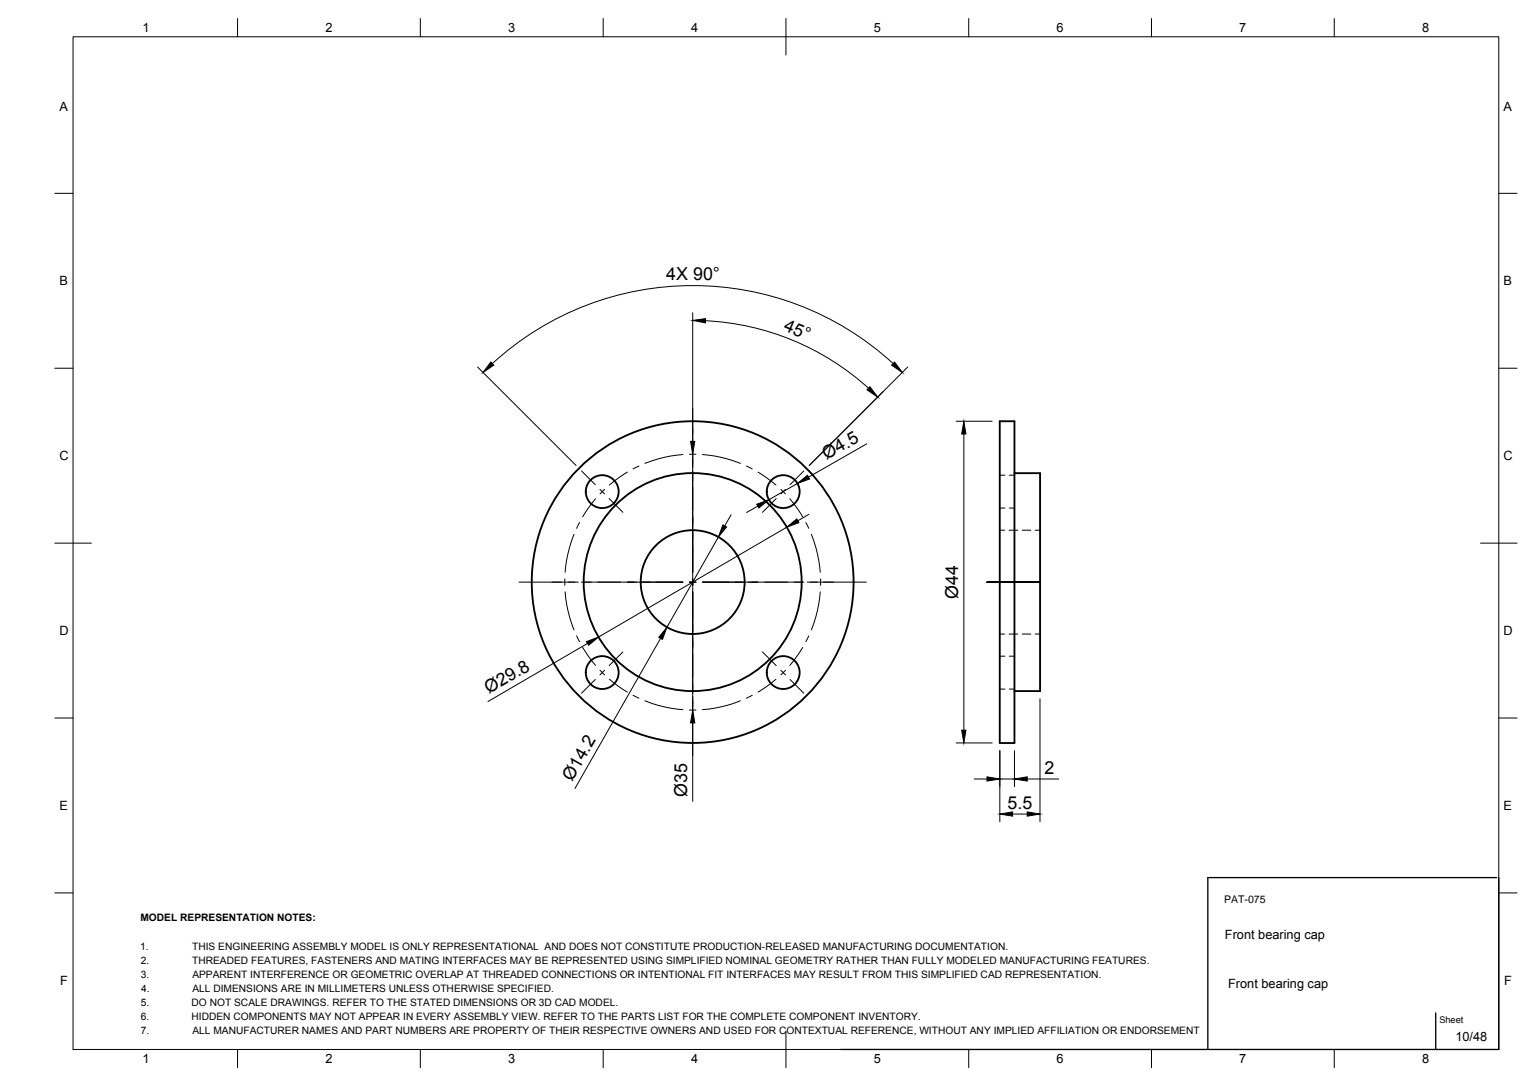
ISO-10303-21;
HEADER;
/* Generated by software containing ST-Developer
 * from STEP Tools, Inc. (www.steptools.com) 
 */

FILE_DESCRIPTION(
/* description */ ('Over-Centre Plunger Toggle Clamp on Slotted Fixture Frame'),
/* implementation_level */ '2;1');

FILE_NAME(
/* name */ 
'Front bearing cap.step',
/* time_stamp */ '2026-10-28T03:23:24-07:00',
/* author */ (''),
/* organization */ (''),
/* preprocessor_version */ 'ST-DEVELOPER v20.2',
/* originating_system */ 'Autodesk Translation Framework v15.17.0.0',
/* authorisation */ '');

FILE_SCHEMA (('AUTOMOTIVE_DESIGN { 1 0 10303 214 3 1 1 }'));
ENDSEC;

DATA;
#10=MECHANICAL_DESIGN_GEOMETRIC_PRESENTATION_REPRESENTATION('',(#518),#15212);
#434=SHAPE_REPRESENTATION_RELATIONSHIP('SRR','None',#15408,#476);
#476=ADVANCED_BREP_SHAPE_REPRESENTATION('',(#569),#15170);
#518=STYLED_ITEM('',(#15719),#569);
#569=MANIFOLD_SOLID_BREP('Body1',#8250);
#671=FACE_BOUND('',#1717,.T.);
#672=FACE_BOUND('',#1721,.T.);
#673=FACE_BOUND('',#1722,.T.);
#674=FACE_BOUND('',#1723,.T.);
#675=FACE_BOUND('',#1724,.T.);
#676=FACE_BOUND('',#1725,.T.);
#677=FACE_BOUND('',#1727,.T.);
#678=FACE_BOUND('',#1728,.T.);
#679=FACE_BOUND('',#1729,.T.);
#680=FACE_BOUND('',#1730,.T.);
#681=FACE_BOUND('',#1731,.T.);
#827=PLANE('',#8932);
#828=PLANE('',#8939);
#829=PLANE('',#8940);
#1165=FACE_OUTER_BOUND('',#1711,.T.);
#1166=FACE_OUTER_BOUND('',#1712,.T.);
#1167=FACE_OUTER_BOUND('',#1713,.T.);
#1168=FACE_OUTER_BOUND('',#1714,.T.);
#1169=FACE_OUTER_BOUND('',#1715,.T.);
#1170=FACE_OUTER_BOUND('',#1716,.T.);
#1171=FACE_OUTER_BOUND('',#1718,.T.);
#1172=FACE_OUTER_BOUND('',#1719,.T.);
#1173=FACE_OUTER_BOUND('',#1720,.T.);
#1174=FACE_OUTER_BOUND('',#1726,.T.);
#1711=EDGE_LOOP('',(#5941,#5942,#5943,#5944));
#1712=EDGE_LOOP('',(#5945,#5946,#5947,#5948));
#1713=EDGE_LOOP('',(#5949,#5950,#5951,#5952));
#1714=EDGE_LOOP('',(#5953,#5954,#5955,#5956));
#1715=EDGE_LOOP('',(#5957,#5958,#5959,#5960));
#1716=EDGE_LOOP('',(#5961));
#1717=EDGE_LOOP('',(#5962));
#1718=EDGE_LOOP('',(#5963,#5964,#5965,#5966));
#1719=EDGE_LOOP('',(#5967,#5968,#5969,#5970));
#1720=EDGE_LOOP('',(#5971));
#1721=EDGE_LOOP('',(#5972));
#1722=EDGE_LOOP('',(#5973));
#1723=EDGE_LOOP('',(#5974));
#1724=EDGE_LOOP('',(#5975));
#1725=EDGE_LOOP('',(#5976));
#1726=EDGE_LOOP('',(#5977));
#1727=EDGE_LOOP('',(#5978));
#1728=EDGE_LOOP('',(#5979));
#1729=EDGE_LOOP('',(#5980));
#1730=EDGE_LOOP('',(#5981));
#1731=EDGE_LOOP('',(#5982));
#2349=LINE('',#12766,#2979);
#2350=LINE('',#12772,#2980);
#2351=LINE('',#12778,#2981);
#2352=LINE('',#12784,#2982);
#2353=LINE('',#12790,#2983);
#2354=LINE('',#12797,#2984);
#2355=LINE('',#12803,#2985);
#2979=VECTOR('',#10184,0.225);
#2980=VECTOR('',#10191,0.225);
#2981=VECTOR('',#10198,0.225);
#2982=VECTOR('',#10205,0.225);
#2983=VECTOR('',#10212,1.49);
#2984=VECTOR('',#10221,0.71);
#2985=VECTOR('',#10228,2.2);
#3559=CIRCLE('',#8918,0.225);
#3560=CIRCLE('',#8919,0.225);
#3561=CIRCLE('',#8921,0.225);
#3562=CIRCLE('',#8922,0.225);
#3563=CIRCLE('',#8924,0.225);
#3564=CIRCLE('',#8925,0.225);
#3565=CIRCLE('',#8927,0.225);
#3566=CIRCLE('',#8928,0.225);
#3567=CIRCLE('',#8930,1.49);
#3568=CIRCLE('',#8931,1.49);
#3569=CIRCLE('',#8933,0.71);
#3570=CIRCLE('',#8935,0.71);
#3571=CIRCLE('',#8937,2.2);
#3572=CIRCLE('',#8938,2.2);
#3983=VERTEX_POINT('',#12763);
#3984=VERTEX_POINT('',#12765);
#3985=VERTEX_POINT('',#12769);
#3986=VERTEX_POINT('',#12771);
#3987=VERTEX_POINT('',#12775);
#3988=VERTEX_POINT('',#12777);
#3989=VERTEX_POINT('',#12781);
#3990=VERTEX_POINT('',#12783);
#3991=VERTEX_POINT('',#12787);
#3992=VERTEX_POINT('',#12789);
#3993=VERTEX_POINT('',#12793);
#3994=VERTEX_POINT('',#12796);
#3995=VERTEX_POINT('',#12800);
#3996=VERTEX_POINT('',#12802);
#4731=EDGE_CURVE('',#3983,#3983,#3559,.T.);
#4732=EDGE_CURVE('',#3983,#3984,#2349,.T.);
#4733=EDGE_CURVE('',#3984,#3984,#3560,.T.);
#4734=EDGE_CURVE('',#3985,#3985,#3561,.T.);
#4735=EDGE_CURVE('',#3985,#3986,#2350,.T.);
#4736=EDGE_CURVE('',#3986,#3986,#3562,.T.);
#4737=EDGE_CURVE('',#3987,#3987,#3563,.T.);
#4738=EDGE_CURVE('',#3987,#3988,#2351,.T.);
#4739=EDGE_CURVE('',#3988,#3988,#3564,.T.);
#4740=EDGE_CURVE('',#3989,#3989,#3565,.T.);
#4741=EDGE_CURVE('',#3989,#3990,#2352,.T.);
#4742=EDGE_CURVE('',#3990,#3990,#3566,.T.);
#4743=EDGE_CURVE('',#3991,#3991,#3567,.T.);
#4744=EDGE_CURVE('',#3991,#3992,#2353,.T.);
#4745=EDGE_CURVE('',#3992,#3992,#3568,.T.);
#4746=EDGE_CURVE('',#3993,#3993,#3569,.T.);
#4747=EDGE_CURVE('',#3993,#3994,#2354,.T.);
#4748=EDGE_CURVE('',#3994,#3994,#3570,.T.);
#4749=EDGE_CURVE('',#3995,#3995,#3571,.T.);
#4750=EDGE_CURVE('',#3995,#3996,#2355,.T.);
#4751=EDGE_CURVE('',#3996,#3996,#3572,.T.);
#5941=ORIENTED_EDGE('',*,*,#4731,.F.);
#5942=ORIENTED_EDGE('',*,*,#4732,.T.);
#5943=ORIENTED_EDGE('',*,*,#4733,.F.);
#5944=ORIENTED_EDGE('',*,*,#4732,.F.);
#5945=ORIENTED_EDGE('',*,*,#4734,.F.);
#5946=ORIENTED_EDGE('',*,*,#4735,.T.);
#5947=ORIENTED_EDGE('',*,*,#4736,.F.);
#5948=ORIENTED_EDGE('',*,*,#4735,.F.);
#5949=ORIENTED_EDGE('',*,*,#4737,.F.);
#5950=ORIENTED_EDGE('',*,*,#4738,.T.);
#5951=ORIENTED_EDGE('',*,*,#4739,.F.);
#5952=ORIENTED_EDGE('',*,*,#4738,.F.);
#5953=ORIENTED_EDGE('',*,*,#4740,.F.);
#5954=ORIENTED_EDGE('',*,*,#4741,.T.);
#5955=ORIENTED_EDGE('',*,*,#4742,.F.);
#5956=ORIENTED_EDGE('',*,*,#4741,.F.);
#5957=ORIENTED_EDGE('',*,*,#4743,.F.);
#5958=ORIENTED_EDGE('',*,*,#4744,.T.);
#5959=ORIENTED_EDGE('',*,*,#4745,.F.);
#5960=ORIENTED_EDGE('',*,*,#4744,.F.);
#5961=ORIENTED_EDGE('',*,*,#4743,.T.);
#5962=ORIENTED_EDGE('',*,*,#4746,.T.);
#5963=ORIENTED_EDGE('',*,*,#4746,.F.);
#5964=ORIENTED_EDGE('',*,*,#4747,.T.);
#5965=ORIENTED_EDGE('',*,*,#4748,.T.);
#5966=ORIENTED_EDGE('',*,*,#4747,.F.);
#5967=ORIENTED_EDGE('',*,*,#4749,.F.);
#5968=ORIENTED_EDGE('',*,*,#4750,.T.);
#5969=ORIENTED_EDGE('',*,*,#4751,.T.);
#5970=ORIENTED_EDGE('',*,*,#4750,.F.);
#5971=ORIENTED_EDGE('',*,*,#4749,.T.);
#5972=ORIENTED_EDGE('',*,*,#4745,.T.);
#5973=ORIENTED_EDGE('',*,*,#4742,.T.);
#5974=ORIENTED_EDGE('',*,*,#4739,.T.);
#5975=ORIENTED_EDGE('',*,*,#4736,.T.);
#5976=ORIENTED_EDGE('',*,*,#4733,.T.);
#5977=ORIENTED_EDGE('',*,*,#4751,.F.);
#5978=ORIENTED_EDGE('',*,*,#4748,.F.);
#5979=ORIENTED_EDGE('',*,*,#4740,.T.);
#5980=ORIENTED_EDGE('',*,*,#4737,.T.);
#5981=ORIENTED_EDGE('',*,*,#4734,.T.);
#5982=ORIENTED_EDGE('',*,*,#4731,.T.);
#7651=CYLINDRICAL_SURFACE('',#8917,0.225);
#7652=CYLINDRICAL_SURFACE('',#8920,0.225);
#7653=CYLINDRICAL_SURFACE('',#8923,0.225);
#7654=CYLINDRICAL_SURFACE('',#8926,0.225);
#7655=CYLINDRICAL_SURFACE('',#8929,1.49);
#7656=CYLINDRICAL_SURFACE('',#8934,0.71);
#7657=CYLINDRICAL_SURFACE('',#8936,2.2);
#7837=ADVANCED_FACE('',(#1165),#7651,.F.);
#7838=ADVANCED_FACE('',(#1166),#7652,.F.);
#7839=ADVANCED_FACE('',(#1167),#7653,.F.);
#7840=ADVANCED_FACE('',(#1168),#7654,.F.);
#7841=ADVANCED_FACE('',(#1169),#7655,.T.);
#7842=ADVANCED_FACE('',(#1170,#671),#827,.T.);
#7843=ADVANCED_FACE('',(#1171),#7656,.F.);
#7844=ADVANCED_FACE('',(#1172),#7657,.T.);
#7845=ADVANCED_FACE('',(#1173,#672,#673,#674,#675,#676),#828,.T.);
#7846=ADVANCED_FACE('',(#1174,#677,#678,#679,#680,#681),#829,.F.);
#8250=CLOSED_SHELL('',(#7837,#7838,#7839,#7840,#7841,#7842,#7843,#7844,
#7845,#7846));
#8916=AXIS2_PLACEMENT_3D('',#12761,#10178,#10179);
#8917=AXIS2_PLACEMENT_3D('',#12762,#10180,#10181);
#8918=AXIS2_PLACEMENT_3D('',#12764,#10182,#10183);
#8919=AXIS2_PLACEMENT_3D('',#12767,#10185,#10186);
#8920=AXIS2_PLACEMENT_3D('',#12768,#10187,#10188);
#8921=AXIS2_PLACEMENT_3D('',#12770,#10189,#10190);
#8922=AXIS2_PLACEMENT_3D('',#12773,#10192,#10193);
#8923=AXIS2_PLACEMENT_3D('',#12774,#10194,#10195);
#8924=AXIS2_PLACEMENT_3D('',#12776,#10196,#10197);
#8925=AXIS2_PLACEMENT_3D('',#12779,#10199,#10200);
#8926=AXIS2_PLACEMENT_3D('',#12780,#10201,#10202);
#8927=AXIS2_PLACEMENT_3D('',#12782,#10203,#10204);
#8928=AXIS2_PLACEMENT_3D('',#12785,#10206,#10207);
#8929=AXIS2_PLACEMENT_3D('',#12786,#10208,#10209);
#8930=AXIS2_PLACEMENT_3D('',#12788,#10210,#10211);
#8931=AXIS2_PLACEMENT_3D('',#12791,#10213,#10214);
#8932=AXIS2_PLACEMENT_3D('',#12792,#10215,#10216);
#8933=AXIS2_PLACEMENT_3D('',#12794,#10217,#10218);
#8934=AXIS2_PLACEMENT_3D('',#12795,#10219,#10220);
#8935=AXIS2_PLACEMENT_3D('',#12798,#10222,#10223);
#8936=AXIS2_PLACEMENT_3D('',#12799,#10224,#10225);
#8937=AXIS2_PLACEMENT_3D('',#12801,#10226,#10227);
#8938=AXIS2_PLACEMENT_3D('',#12804,#10229,#10230);
#8939=AXIS2_PLACEMENT_3D('',#12805,#10231,#10232);
#8940=AXIS2_PLACEMENT_3D('',#12806,#10233,#10234);
#10178=DIRECTION('axis',(0.,0.,1.));
#10179=DIRECTION('refdir',(1.,0.,0.));
#10180=DIRECTION('center_axis',(0.,1.,0.));
#10181=DIRECTION('ref_axis',(1.,0.,0.));
#10182=DIRECTION('center_axis',(0.,1.,0.));
#10183=DIRECTION('ref_axis',(1.,0.,0.));
#10184=DIRECTION('',(0.,1.,0.));
#10185=DIRECTION('center_axis',(0.,-1.,0.));
#10186=DIRECTION('ref_axis',(1.,0.,0.));
#10187=DIRECTION('center_axis',(0.,1.,0.));
#10188=DIRECTION('ref_axis',(1.,0.,0.));
#10189=DIRECTION('center_axis',(0.,1.,0.));
#10190=DIRECTION('ref_axis',(1.,0.,0.));
#10191=DIRECTION('',(0.,1.,0.));
#10192=DIRECTION('center_axis',(0.,-1.,0.));
#10193=DIRECTION('ref_axis',(1.,0.,0.));
#10194=DIRECTION('center_axis',(0.,1.,0.));
#10195=DIRECTION('ref_axis',(1.,0.,0.));
#10196=DIRECTION('center_axis',(0.,1.,0.));
#10197=DIRECTION('ref_axis',(1.,0.,0.));
#10198=DIRECTION('',(0.,1.,0.));
#10199=DIRECTION('center_axis',(0.,-1.,0.));
#10200=DIRECTION('ref_axis',(1.,0.,0.));
#10201=DIRECTION('center_axis',(0.,1.,0.));
#10202=DIRECTION('ref_axis',(1.,0.,0.));
#10203=DIRECTION('center_axis',(0.,1.,0.));
#10204=DIRECTION('ref_axis',(1.,0.,0.));
#10205=DIRECTION('',(0.,1.,0.));
#10206=DIRECTION('center_axis',(0.,-1.,0.));
#10207=DIRECTION('ref_axis',(1.,0.,0.));
#10208=DIRECTION('center_axis',(0.,1.,0.));
#10209=DIRECTION('ref_axis',(1.,0.,0.));
#10210=DIRECTION('center_axis',(0.,1.,0.));
#10211=DIRECTION('ref_axis',(1.,0.,0.));
#10212=DIRECTION('',(0.,-1.,0.));
#10213=DIRECTION('center_axis',(0.,-1.,0.));
#10214=DIRECTION('ref_axis',(1.,0.,0.));
#10215=DIRECTION('center_axis',(0.,1.,0.));
#10216=DIRECTION('ref_axis',(1.,0.,0.));
#10217=DIRECTION('center_axis',(0.,-1.,0.));
#10218=DIRECTION('ref_axis',(1.,0.,0.));
#10219=DIRECTION('center_axis',(0.,1.,0.));
#10220=DIRECTION('ref_axis',(1.,0.,0.));
#10221=DIRECTION('',(0.,-1.,0.));
#10222=DIRECTION('center_axis',(0.,-1.,0.));
#10223=DIRECTION('ref_axis',(1.,0.,0.));
#10224=DIRECTION('center_axis',(0.,1.,0.));
#10225=DIRECTION('ref_axis',(1.,0.,0.));
#10226=DIRECTION('center_axis',(0.,1.,0.));
#10227=DIRECTION('ref_axis',(1.,0.,0.));
#10228=DIRECTION('',(0.,-1.,0.));
#10229=DIRECTION('center_axis',(0.,1.,0.));
#10230=DIRECTION('ref_axis',(1.,0.,0.));
#10231=DIRECTION('center_axis',(0.,1.,0.));
#10232=DIRECTION('ref_axis',(1.,0.,0.));
#10233=DIRECTION('center_axis',(0.,1.,0.));
#10234=DIRECTION('ref_axis',(1.,0.,0.));
#12761=CARTESIAN_POINT('',(0.,0.,0.));
#12762=CARTESIAN_POINT('Origin',(-5.23743686707646,-1.1,9.76256313292354));
#12763=CARTESIAN_POINT('',(-5.46243686707646,-1.,9.76256313292354));
#12764=CARTESIAN_POINT('Origin',(-5.23743686707646,-1.,9.76256313292354));
#12765=CARTESIAN_POINT('',(-5.46243686707646,-0.8,9.76256313292354));
#12766=CARTESIAN_POINT('',(-5.46243686707646,-1.1,9.76256313292354));
#12767=CARTESIAN_POINT('Origin',(-5.23743686707646,-0.8,9.76256313292354));
#12768=CARTESIAN_POINT('Origin',(-5.23743686707646,-1.1,12.2374368670765));
#12769=CARTESIAN_POINT('',(-5.46243686707646,-1.,12.2374368670765));
#12770=CARTESIAN_POINT('Origin',(-5.23743686707646,-1.,12.2374368670765));
#12771=CARTESIAN_POINT('',(-5.46243686707646,-0.8,12.2374368670765));
#12772=CARTESIAN_POINT('',(-5.46243686707646,-1.1,12.2374368670765));
#12773=CARTESIAN_POINT('Origin',(-5.23743686707646,-0.8,12.2374368670765));
#12774=CARTESIAN_POINT('Origin',(-2.76256313292354,-1.1,12.2374368670765));
#12775=CARTESIAN_POINT('',(-2.98756313292354,-1.,12.2374368670765));
#12776=CARTESIAN_POINT('Origin',(-2.76256313292354,-1.,12.2374368670765));
#12777=CARTESIAN_POINT('',(-2.98756313292354,-0.8,12.2374368670765));
#12778=CARTESIAN_POINT('',(-2.98756313292354,-1.1,12.2374368670765));
#12779=CARTESIAN_POINT('Origin',(-2.76256313292354,-0.8,12.2374368670765));
#12780=CARTESIAN_POINT('Origin',(-2.76256313292354,-1.1,9.76256313292354));
#12781=CARTESIAN_POINT('',(-2.98756313292354,-1.,9.76256313292354));
#12782=CARTESIAN_POINT('Origin',(-2.76256313292354,-1.,9.76256313292354));
#12783=CARTESIAN_POINT('',(-2.98756313292354,-0.8,9.76256313292354));
#12784=CARTESIAN_POINT('',(-2.98756313292354,-1.1,9.76256313292354));
#12785=CARTESIAN_POINT('Origin',(-2.76256313292354,-0.8,9.76256313292354));
#12786=CARTESIAN_POINT('Origin',(-4.,-0.8,11.));
#12787=CARTESIAN_POINT('',(-5.49,-0.45,11.));
#12788=CARTESIAN_POINT('Origin',(-4.,-0.45,11.));
#12789=CARTESIAN_POINT('',(-5.49,-0.8,11.));
#12790=CARTESIAN_POINT('',(-5.49,-0.8,11.));
#12791=CARTESIAN_POINT('Origin',(-4.,-0.8,11.));
#12792=CARTESIAN_POINT('Origin',(-4.,-0.45,11.));
#12793=CARTESIAN_POINT('',(-4.71,-0.45,11.));
#12794=CARTESIAN_POINT('Origin',(-4.,-0.45,11.));
#12795=CARTESIAN_POINT('Origin',(-4.,-1.,11.));
#12796=CARTESIAN_POINT('',(-4.71,-1.,11.));
#12797=CARTESIAN_POINT('',(-4.71,-1.,11.));
#12798=CARTESIAN_POINT('Origin',(-4.,-1.,11.));
#12799=CARTESIAN_POINT('Origin',(-4.,-1.,11.));
#12800=CARTESIAN_POINT('',(-6.2,-0.8,11.));
#12801=CARTESIAN_POINT('Origin',(-4.,-0.8,11.));
#12802=CARTESIAN_POINT('',(-6.2,-1.,11.));
#12803=CARTESIAN_POINT('',(-6.2,-1.,11.));
#12804=CARTESIAN_POINT('Origin',(-4.,-1.,11.));
#12805=CARTESIAN_POINT('Origin',(-4.,-0.8,11.));
#12806=CARTESIAN_POINT('Origin',(-4.,-1.,11.));
#15120=UNCERTAINTY_MEASURE_WITH_UNIT(LENGTH_MEASURE(0.001),#15213,
'DISTANCE_ACCURACY_VALUE',
'Maximum model space distance between geometric entities at asserted c
onnectivities');
#15162=UNCERTAINTY_MEASURE_WITH_UNIT(LENGTH_MEASURE(0.001),#15213,
'DISTANCE_ACCURACY_VALUE',
'Maximum model space distance between geometric entities at asserted c
onnectivities');
#15170=(
GEOMETRIC_REPRESENTATION_CONTEXT(3)
GLOBAL_UNCERTAINTY_ASSIGNED_CONTEXT((#15120))
GLOBAL_UNIT_ASSIGNED_CONTEXT((#15213,#15215,#15216))
REPRESENTATION_CONTEXT('','3D')
);
#15212=(
GEOMETRIC_REPRESENTATION_CONTEXT(3)
GLOBAL_UNCERTAINTY_ASSIGNED_CONTEXT((#15162))
GLOBAL_UNIT_ASSIGNED_CONTEXT((#15213,#15215,#15216))
REPRESENTATION_CONTEXT('','3D')
);
#15213=(
LENGTH_UNIT()
NAMED_UNIT(*)
SI_UNIT(.CENTI.,.METRE.)
);
#15215=(
NAMED_UNIT(*)
PLANE_ANGLE_UNIT()
SI_UNIT($,.RADIAN.)
);
#15216=(
NAMED_UNIT(*)
SI_UNIT($,.STERADIAN.)
SOLID_ANGLE_UNIT()
);
#15224=SHAPE_DEFINITION_REPRESENTATION(#15273,#15408);
#15273=PRODUCT_DEFINITION_SHAPE('',$,#15458);
#15408=SHAPE_REPRESENTATION('',(#8916),#15170);
#15450=PRODUCT_DEFINITION_CONTEXT('part definition',#15599,'design');
#15458=PRODUCT_DEFINITION('Front bearing cap','Front bearing cap',#15507,
#15450);
#15507=PRODUCT_DEFINITION_FORMATION('',$,#15608);
#15599=APPLICATION_CONTEXT(
'Core Data for Automotive Mechanical Design Process');
#15600=PRODUCT_CONTEXT('part definition',#15599,'mechanical');
#15608=PRODUCT('Front bearing cap','Front bearing cap',
'Front bearing cap',(#15600));
#15713=COLOUR_RGB('Grey',0.48,0.52,0.57);
#15714=FILL_AREA_STYLE_COLOUR('',#15713);
#15715=FILL_AREA_STYLE('',(#15714));
#15716=SURFACE_STYLE_FILL_AREA(#15715);
#15717=SURFACE_SIDE_STYLE('',(#15716));
#15718=SURFACE_STYLE_USAGE(.BOTH.,#15717);
#15719=PRESENTATION_STYLE_ASSIGNMENT((#15718));
ENDSEC;
END-ISO-10303-21;
